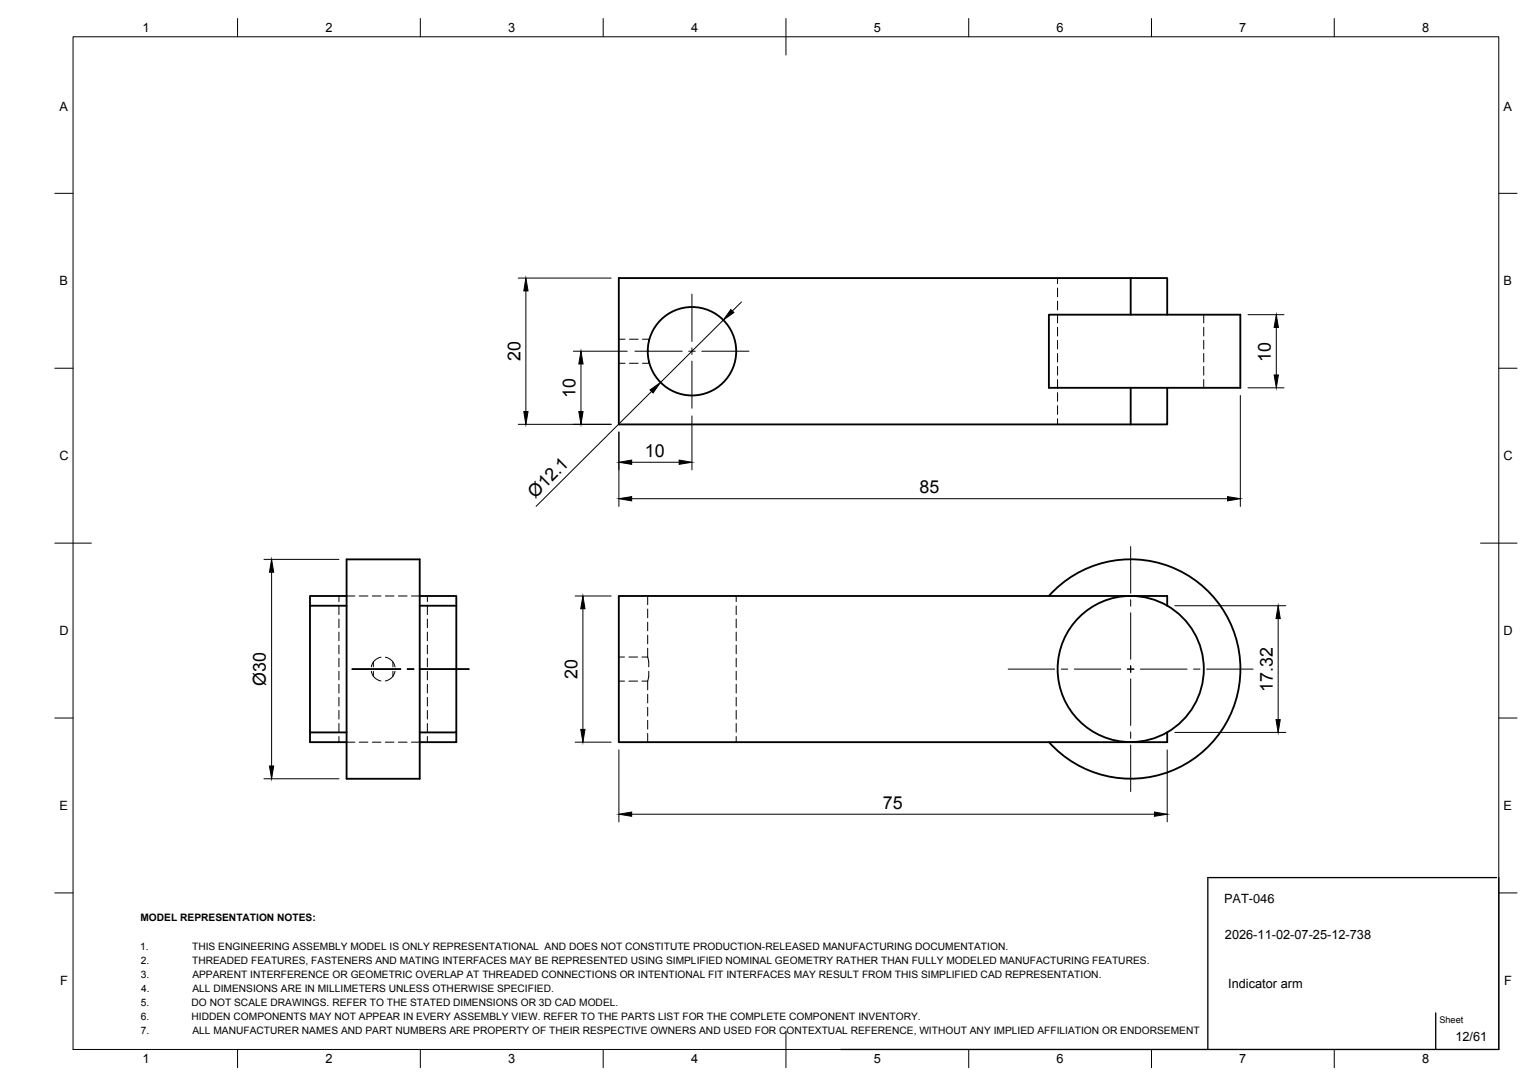
ISO-10303-21;
HEADER;
/* Generated by software containing ST-Developer
 * from STEP Tools, Inc. (www.steptools.com) 
 */

FILE_DESCRIPTION(
/* description */ ('Gear mesh backlash fixture'),
/* implementation_level */ '2;1');

FILE_NAME(
/* name */ 'Indicator arm.step',
/* time_stamp */ '2026-10-28T03:26:00-07:00',
/* author */ (''),
/* organization */ (''),
/* preprocessor_version */ 'ST-DEVELOPER v20.2',
/* originating_system */ 'Autodesk Translation Framework v15.17.0.0',
/* authorisation */ '');

FILE_SCHEMA (('AUTOMOTIVE_DESIGN { 1 0 10303 214 3 1 1 }'));
ENDSEC;

DATA;
#10=MECHANICAL_DESIGN_GEOMETRIC_PRESENTATION_REPRESENTATION('',(#1023),#57900);
#788=B_SPLINE_CURVE_WITH_KNOTS('',3,(#19722,#19723,#19724,#19725,#19726,
#19727,#19728,#19729,#19730,#19731,#19732,#19733,#19734,#19735),
 .UNSPECIFIED.,.F.,.F.,(4,2,2,2,2,2,4),(0.598759573717661,0.624973342427789,
0.687463163426142,0.749952984424494,0.812442805422847,0.874932626421199,
0.901146395131325),.UNSPECIFIED.);
#789=B_SPLINE_CURVE_WITH_KNOTS('',3,(#19739,#19740,#19741,#19742,#19743,
#19744,#19745,#19746),.UNSPECIFIED.,.F.,.F.,(4,2,2,4),(0.249984328141498,
0.31247414913985,0.374963970138203,0.401177738848332),.UNSPECIFIED.);
#790=B_SPLINE_CURVE_WITH_KNOTS('',3,(#19750,#19751,#19752,#19753,#19754,
#19755,#19756,#19757),.UNSPECIFIED.,.F.,.F.,(4,2,2,4),(0.0987909174346634,
0.125004686144793,0.187494507143146,0.249984328141498),.UNSPECIFIED.);
#923=SHAPE_REPRESENTATION_RELATIONSHIP('SRR','None',#58118,#973);
#973=ADVANCED_BREP_SHAPE_REPRESENTATION('',(#1088),#57851);
#1023=STYLED_ITEM('',(#58451),#1088);
#1088=MANIFOLD_SOLID_BREP('Body1',#13583);
#1199=FACE_BOUND('',#2617,.T.);
#1200=FACE_BOUND('',#2619,.T.);
#1201=FACE_BOUND('',#2625,.T.);
#1202=FACE_BOUND('',#2628,.T.);
#1368=PLANE('',#14390);
#1369=PLANE('',#14395);
#1370=PLANE('',#14407);
#1371=PLANE('',#14409);
#1372=PLANE('',#14410);
#1373=PLANE('',#14411);
#1374=PLANE('',#14412);
#1375=PLANE('',#14413);
#1376=PLANE('',#14414);
#1377=PLANE('',#14415);
#1378=PLANE('',#14416);
#1379=PLANE('',#14417);
#1380=PLANE('',#14418);
#1381=PLANE('',#14419);
#1382=PLANE('',#14420);
#1383=PLANE('',#14426);
#1384=PLANE('',#14427);
#1385=PLANE('',#14428);
#1386=PLANE('',#14429);
#1387=PLANE('',#14430);
#1388=PLANE('',#14431);
#1779=FACE_OUTER_BOUND('',#2600,.T.);
#1780=FACE_OUTER_BOUND('',#2601,.T.);
#1781=FACE_OUTER_BOUND('',#2602,.T.);
#1782=FACE_OUTER_BOUND('',#2603,.T.);
#1783=FACE_OUTER_BOUND('',#2604,.T.);
#1784=FACE_OUTER_BOUND('',#2605,.T.);
#1785=FACE_OUTER_BOUND('',#2606,.T.);
#1786=FACE_OUTER_BOUND('',#2607,.T.);
#1787=FACE_OUTER_BOUND('',#2608,.T.);
#1788=FACE_OUTER_BOUND('',#2609,.T.);
#1789=FACE_OUTER_BOUND('',#2610,.T.);
#1790=FACE_OUTER_BOUND('',#2611,.T.);
#1791=FACE_OUTER_BOUND('',#2612,.T.);
#1792=FACE_OUTER_BOUND('',#2613,.T.);
#1793=FACE_OUTER_BOUND('',#2614,.T.);
#1794=FACE_OUTER_BOUND('',#2615,.T.);
#1795=FACE_OUTER_BOUND('',#2616,.T.);
#1796=FACE_OUTER_BOUND('',#2618,.T.);
#1797=FACE_OUTER_BOUND('',#2620,.T.);
#1798=FACE_OUTER_BOUND('',#2621,.T.);
#1799=FACE_OUTER_BOUND('',#2622,.T.);
#1800=FACE_OUTER_BOUND('',#2623,.T.);
#1801=FACE_OUTER_BOUND('',#2624,.T.);
#1802=FACE_OUTER_BOUND('',#2626,.T.);
#1803=FACE_OUTER_BOUND('',#2627,.T.);
#2600=EDGE_LOOP('',(#9261,#9262));
#2601=EDGE_LOOP('',(#9263,#9264,#9265,#9266,#9267,#9268,#9269,#9270));
#2602=EDGE_LOOP('',(#9271,#9272));
#2603=EDGE_LOOP('',(#9273,#9274,#9275,#9276,#9277,#9278,#9279,#9280,#9281,
#9282,#9283,#9284,#9285,#9286,#9287,#9288,#9289,#9290,#9291,#9292,#9293,
#9294,#9295,#9296));
#2604=EDGE_LOOP('',(#9297,#9298,#9299,#9300,#9301,#9302,#9303,#9304,#9305));
#2605=EDGE_LOOP('',(#9306,#9307,#9308,#9309));
#2606=EDGE_LOOP('',(#9310,#9311,#9312));
#2607=EDGE_LOOP('',(#9313,#9314,#9315,#9316));
#2608=EDGE_LOOP('',(#9317,#9318,#9319,#9320));
#2609=EDGE_LOOP('',(#9321,#9322,#9323,#9324));
#2610=EDGE_LOOP('',(#9325,#9326,#9327,#9328));
#2611=EDGE_LOOP('',(#9329,#9330,#9331,#9332));
#2612=EDGE_LOOP('',(#9333,#9334,#9335,#9336));
#2613=EDGE_LOOP('',(#9337,#9338,#9339));
#2614=EDGE_LOOP('',(#9340,#9341,#9342));
#2615=EDGE_LOOP('',(#9343,#9344,#9345,#9346));
#2616=EDGE_LOOP('',(#9347,#9348,#9349,#9350,#9351,#9352,#9353,#9354));
#2617=EDGE_LOOP('',(#9355));
#2618=EDGE_LOOP('',(#9356,#9357,#9358,#9359));
#2619=EDGE_LOOP('',(#9360,#9361,#9362,#9363,#9364));
#2620=EDGE_LOOP('',(#9365,#9366,#9367,#9368));
#2621=EDGE_LOOP('',(#9369,#9370,#9371,#9372,#9373,#9374,#9375,#9376,#9377));
#2622=EDGE_LOOP('',(#9378,#9379,#9380,#9381));
#2623=EDGE_LOOP('',(#9382,#9383,#9384,#9385));
#2624=EDGE_LOOP('',(#9386,#9387,#9388,#9389));
#2625=EDGE_LOOP('',(#9390));
#2626=EDGE_LOOP('',(#9391,#9392,#9393));
#2627=EDGE_LOOP('',(#9394,#9395,#9396,#9397,#9398,#9399,#9400,#9401));
#2628=EDGE_LOOP('',(#9402));
#3498=LINE('',#19718,#4387);
#3499=LINE('',#19748,#4388);
#3500=LINE('',#19759,#4389);
#3501=LINE('',#19763,#4390);
#3502=LINE('',#19767,#4391);
#3503=LINE('',#19771,#4392);
#3504=LINE('',#19775,#4393);
#3505=LINE('',#19779,#4394);
#3506=LINE('',#19780,#4395);
#3507=LINE('',#19784,#4396);
#3508=LINE('',#19785,#4397);
#3509=LINE('',#19789,#4398);
#3510=LINE('',#19794,#4399);
#3511=LINE('',#19798,#4400);
#3512=LINE('',#19799,#4401);
#3513=LINE('',#19801,#4402);
#3514=LINE('',#19804,#4403);
#3515=LINE('',#19805,#4404);
#3516=LINE('',#19807,#4405);
#3517=LINE('',#19810,#4406);
#3518=LINE('',#19812,#4407);
#3519=LINE('',#19813,#4408);
#3520=LINE('',#19816,#4409);
#3521=LINE('',#19817,#4410);
#3522=LINE('',#19819,#4411);
#3523=LINE('',#19822,#4412);
#3524=LINE('',#19824,#4413);
#3525=LINE('',#19825,#4414);
#3526=LINE('',#19828,#4415);
#3527=LINE('',#19830,#4416);
#3528=LINE('',#19831,#4417);
#3529=LINE('',#19834,#4418);
#3530=LINE('',#19835,#4419);
#3531=LINE('',#19838,#4420);
#3532=LINE('',#19840,#4421);
#3533=LINE('',#19841,#4422);
#3534=LINE('',#19843,#4423);
#3535=LINE('',#19844,#4424);
#3536=LINE('',#19847,#4425);
#3537=LINE('',#19849,#4426);
#3538=LINE('',#19850,#4427);
#3539=LINE('',#19852,#4428);
#3540=LINE('',#19855,#4429);
#3541=LINE('',#19857,#4430);
#3542=LINE('',#19859,#4431);
#3543=LINE('',#19860,#4432);
#3544=LINE('',#19866,#4433);
#3545=LINE('',#19869,#4434);
#3546=LINE('',#19872,#4435);
#3547=LINE('',#19875,#4436);
#3548=LINE('',#19877,#4437);
#4387=VECTOR('',#16057,1.);
#4388=VECTOR('',#16064,0.164999999999999);
#4389=VECTOR('',#16069,1.);
#4390=VECTOR('',#16072,1.);
#4391=VECTOR('',#16075,1.);
#4392=VECTOR('',#16078,1.);
#4393=VECTOR('',#16081,1.);
#4394=VECTOR('',#16084,1.);
#4395=VECTOR('',#16085,1.);
#4396=VECTOR('',#16088,1.);
#4397=VECTOR('',#16089,1.);
#4398=VECTOR('',#16092,1.);
#4399=VECTOR('',#16097,1.);
#4400=VECTOR('',#16100,1.);
#4401=VECTOR('',#16101,1.);
#4402=VECTOR('',#16104,1.);
#4403=VECTOR('',#16107,1.);
#4404=VECTOR('',#16108,1.);
#4405=VECTOR('',#16109,1.);
#4406=VECTOR('',#16112,1.);
#4407=VECTOR('',#16113,1.);
#4408=VECTOR('',#16114,1.);
#4409=VECTOR('',#16117,1.);
#4410=VECTOR('',#16118,1.);
#4411=VECTOR('',#16121,1.);
#4412=VECTOR('',#16124,1.);
#4413=VECTOR('',#16125,1.);
#4414=VECTOR('',#16126,1.);
#4415=VECTOR('',#16129,1.);
#4416=VECTOR('',#16130,1.);
#4417=VECTOR('',#16131,1.);
#4418=VECTOR('',#16134,1.);
#4419=VECTOR('',#16135,1.);
#4420=VECTOR('',#16138,1.);
#4421=VECTOR('',#16139,1.);
#4422=VECTOR('',#16140,1.);
#4423=VECTOR('',#16143,1.);
#4424=VECTOR('',#16144,1.);
#4425=VECTOR('',#16147,1.);
#4426=VECTOR('',#16148,1.);
#4427=VECTOR('',#16149,1.);
#4428=VECTOR('',#16152,1.);
#4429=VECTOR('',#16157,1.);
#4430=VECTOR('',#16160,1.);
#4431=VECTOR('',#16161,1.);
#4432=VECTOR('',#16162,1.);
#4433=VECTOR('',#16169,0.605);
#4434=VECTOR('',#16172,1.);
#4435=VECTOR('',#16177,1.);
#4436=VECTOR('',#16182,1.);
#4437=VECTOR('',#16185,1.);
#5289=CIRCLE('',#14391,0.164999999999999);
#5290=CIRCLE('',#14393,0.164999999999999);
#5291=CIRCLE('',#14394,0.164999999999999);
#5292=CIRCLE('',#14397,1.);
#5293=CIRCLE('',#14398,1.);
#5294=CIRCLE('',#14399,1.);
#5295=CIRCLE('',#14400,1.);
#5296=CIRCLE('',#14401,1.);
#5297=CIRCLE('',#14402,1.);
#5298=CIRCLE('',#14403,1.);
#5299=CIRCLE('',#14404,1.);
#5300=CIRCLE('',#14405,1.);
#5301=CIRCLE('',#14406,1.);
#5302=CIRCLE('',#14408,1.5);
#5303=CIRCLE('',#14421,0.605);
#5304=CIRCLE('',#14423,0.605);
#5305=CIRCLE('',#14425,1.5);
#5909=VERTEX_POINT('',#19716);
#5910=VERTEX_POINT('',#19717);
#5911=VERTEX_POINT('',#19721);
#5912=VERTEX_POINT('',#19736);
#5913=VERTEX_POINT('',#19738);
#5914=VERTEX_POINT('',#19747);
#5915=VERTEX_POINT('',#19761);
#5916=VERTEX_POINT('',#19762);
#5917=VERTEX_POINT('',#19764);
#5918=VERTEX_POINT('',#19766);
#5919=VERTEX_POINT('',#19768);
#5920=VERTEX_POINT('',#19770);
#5921=VERTEX_POINT('',#19772);
#5922=VERTEX_POINT('',#19774);
#5923=VERTEX_POINT('',#19776);
#5924=VERTEX_POINT('',#19778);
#5925=VERTEX_POINT('',#19781);
#5926=VERTEX_POINT('',#19783);
#5927=VERTEX_POINT('',#19786);
#5928=VERTEX_POINT('',#19788);
#5929=VERTEX_POINT('',#19791);
#5930=VERTEX_POINT('',#19793);
#5931=VERTEX_POINT('',#19795);
#5932=VERTEX_POINT('',#19797);
#5933=VERTEX_POINT('',#19803);
#5934=VERTEX_POINT('',#19806);
#5935=VERTEX_POINT('',#19808);
#5936=VERTEX_POINT('',#19811);
#5937=VERTEX_POINT('',#19815);
#5938=VERTEX_POINT('',#19821);
#5939=VERTEX_POINT('',#19823);
#5940=VERTEX_POINT('',#19827);
#5941=VERTEX_POINT('',#19829);
#5942=VERTEX_POINT('',#19833);
#5943=VERTEX_POINT('',#19837);
#5944=VERTEX_POINT('',#19839);
#5945=VERTEX_POINT('',#19846);
#5946=VERTEX_POINT('',#19848);
#5947=VERTEX_POINT('',#19858);
#5948=VERTEX_POINT('',#19861);
#5949=VERTEX_POINT('',#19864);
#5950=VERTEX_POINT('',#19868);
#7217=EDGE_CURVE('',#5909,#5910,#3498,.T.);
#7218=EDGE_CURVE('',#5909,#5910,#5289,.T.);
#7219=EDGE_CURVE('',#5911,#5909,#788,.T.);
#7220=EDGE_CURVE('',#5912,#5911,#5290,.T.);
#7221=EDGE_CURVE('',#5913,#5912,#789,.T.);
#7222=EDGE_CURVE('',#5913,#5914,#3499,.T.);
#7223=EDGE_CURVE('',#5914,#5914,#5291,.T.);
#7224=EDGE_CURVE('',#5910,#5913,#790,.T.);
#7225=EDGE_CURVE('',#5912,#5911,#3500,.T.);
#7226=EDGE_CURVE('',#5915,#5916,#3501,.T.);
#7227=EDGE_CURVE('',#5917,#5915,#5292,.T.);
#7228=EDGE_CURVE('',#5918,#5917,#3502,.T.);
#7229=EDGE_CURVE('',#5919,#5918,#5293,.T.);
#7230=EDGE_CURVE('',#5919,#5920,#3503,.T.);
#7231=EDGE_CURVE('',#5921,#5920,#5294,.T.);
#7232=EDGE_CURVE('',#5922,#5921,#3504,.T.);
#7233=EDGE_CURVE('',#5923,#5922,#5295,.T.);
#7234=EDGE_CURVE('',#5924,#5923,#3505,.T.);
#7235=EDGE_CURVE('',#5924,#5923,#3506,.T.);
#7236=EDGE_CURVE('',#5925,#5923,#5296,.T.);
#7237=EDGE_CURVE('',#5926,#5925,#3507,.T.);
#7238=EDGE_CURVE('',#5926,#5925,#3508,.T.);
#7239=EDGE_CURVE('',#5927,#5925,#5297,.T.);
#7240=EDGE_CURVE('',#5928,#5927,#3509,.T.);
#7241=EDGE_CURVE('',#5920,#5928,#5298,.T.);
#7242=EDGE_CURVE('',#5929,#5919,#5299,.T.);
#7243=EDGE_CURVE('',#5930,#5929,#3510,.T.);
#7244=EDGE_CURVE('',#5931,#5930,#5300,.T.);
#7245=EDGE_CURVE('',#5931,#5932,#3511,.T.);
#7246=EDGE_CURVE('',#5931,#5932,#3512,.T.);
#7247=EDGE_CURVE('',#5915,#5931,#5301,.T.);
#7248=EDGE_CURVE('',#5915,#5916,#3513,.T.);
#7249=EDGE_CURVE('',#5933,#5918,#3514,.T.);
#7250=EDGE_CURVE('',#5916,#5933,#3515,.T.);
#7251=EDGE_CURVE('',#5934,#5916,#3516,.T.);
#7252=EDGE_CURVE('',#5935,#5934,#5302,.T.);
#7253=EDGE_CURVE('',#5932,#5935,#3517,.T.);
#7254=EDGE_CURVE('',#5936,#5932,#3518,.T.);
#7255=EDGE_CURVE('',#5929,#5936,#3519,.T.);
#7256=EDGE_CURVE('',#5917,#5937,#3520,.T.);
#7257=EDGE_CURVE('',#5933,#5937,#3521,.T.);
#7258=EDGE_CURVE('',#5937,#5915,#3522,.T.);
#7259=EDGE_CURVE('',#5931,#5938,#3523,.T.);
#7260=EDGE_CURVE('',#5938,#5939,#3524,.T.);
#7261=EDGE_CURVE('',#5915,#5939,#3525,.T.);
#7262=EDGE_CURVE('',#5926,#5940,#3526,.T.);
#7263=EDGE_CURVE('',#5941,#5940,#3527,.T.);
#7264=EDGE_CURVE('',#5925,#5941,#3528,.T.);
#7265=EDGE_CURVE('',#5942,#5931,#3529,.T.);
#7266=EDGE_CURVE('',#5936,#5942,#3530,.T.);
#7267=EDGE_CURVE('',#5921,#5943,#3531,.T.);
#7268=EDGE_CURVE('',#5944,#5943,#3532,.T.);
#7269=EDGE_CURVE('',#5922,#5944,#3533,.T.);
#7270=EDGE_CURVE('',#5941,#5927,#3534,.T.);
#7271=EDGE_CURVE('',#5940,#5928,#3535,.T.);
#7272=EDGE_CURVE('',#5945,#5923,#3536,.T.);
#7273=EDGE_CURVE('',#5946,#5945,#3537,.T.);
#7274=EDGE_CURVE('',#5946,#5925,#3538,.T.);
#7275=EDGE_CURVE('',#5923,#5944,#3539,.T.);
#7276=EDGE_CURVE('',#5943,#5924,#3540,.T.);
#7277=EDGE_CURVE('',#5939,#5945,#3541,.T.);
#7278=EDGE_CURVE('',#5924,#5947,#3542,.T.);
#7279=EDGE_CURVE('',#5947,#5934,#3543,.T.);
#7280=EDGE_CURVE('',#5948,#5948,#5303,.T.);
#7281=EDGE_CURVE('',#5949,#5949,#5304,.T.);
#7282=EDGE_CURVE('',#5949,#5948,#3544,.T.);
#7283=EDGE_CURVE('',#5935,#5950,#3545,.T.);
#7284=EDGE_CURVE('',#5950,#5947,#5305,.T.);
#7285=EDGE_CURVE('',#5950,#5926,#3546,.T.);
#7286=EDGE_CURVE('',#5942,#5930,#3547,.T.);
#7287=EDGE_CURVE('',#5938,#5946,#3548,.T.);
#9261=ORIENTED_EDGE('',*,*,#7217,.F.);
#9262=ORIENTED_EDGE('',*,*,#7218,.T.);
#9263=ORIENTED_EDGE('',*,*,#7219,.F.);
#9264=ORIENTED_EDGE('',*,*,#7220,.F.);
#9265=ORIENTED_EDGE('',*,*,#7221,.F.);
#9266=ORIENTED_EDGE('',*,*,#7222,.T.);
#9267=ORIENTED_EDGE('',*,*,#7223,.F.);
#9268=ORIENTED_EDGE('',*,*,#7222,.F.);
#9269=ORIENTED_EDGE('',*,*,#7224,.F.);
#9270=ORIENTED_EDGE('',*,*,#7218,.F.);
#9271=ORIENTED_EDGE('',*,*,#7225,.F.);
#9272=ORIENTED_EDGE('',*,*,#7220,.T.);
#9273=ORIENTED_EDGE('',*,*,#7226,.F.);
#9274=ORIENTED_EDGE('',*,*,#7227,.F.);
#9275=ORIENTED_EDGE('',*,*,#7228,.F.);
#9276=ORIENTED_EDGE('',*,*,#7229,.F.);
#9277=ORIENTED_EDGE('',*,*,#7230,.T.);
#9278=ORIENTED_EDGE('',*,*,#7231,.F.);
#9279=ORIENTED_EDGE('',*,*,#7232,.F.);
#9280=ORIENTED_EDGE('',*,*,#7233,.F.);
#9281=ORIENTED_EDGE('',*,*,#7234,.F.);
#9282=ORIENTED_EDGE('',*,*,#7235,.T.);
#9283=ORIENTED_EDGE('',*,*,#7236,.F.);
#9284=ORIENTED_EDGE('',*,*,#7237,.F.);
#9285=ORIENTED_EDGE('',*,*,#7238,.T.);
#9286=ORIENTED_EDGE('',*,*,#7239,.F.);
#9287=ORIENTED_EDGE('',*,*,#7240,.F.);
#9288=ORIENTED_EDGE('',*,*,#7241,.F.);
#9289=ORIENTED_EDGE('',*,*,#7230,.F.);
#9290=ORIENTED_EDGE('',*,*,#7242,.F.);
#9291=ORIENTED_EDGE('',*,*,#7243,.F.);
#9292=ORIENTED_EDGE('',*,*,#7244,.F.);
#9293=ORIENTED_EDGE('',*,*,#7245,.T.);
#9294=ORIENTED_EDGE('',*,*,#7246,.F.);
#9295=ORIENTED_EDGE('',*,*,#7247,.F.);
#9296=ORIENTED_EDGE('',*,*,#7248,.T.);
#9297=ORIENTED_EDGE('',*,*,#7242,.T.);
#9298=ORIENTED_EDGE('',*,*,#7229,.T.);
#9299=ORIENTED_EDGE('',*,*,#7249,.F.);
#9300=ORIENTED_EDGE('',*,*,#7250,.F.);
#9301=ORIENTED_EDGE('',*,*,#7251,.F.);
#9302=ORIENTED_EDGE('',*,*,#7252,.F.);
#9303=ORIENTED_EDGE('',*,*,#7253,.F.);
#9304=ORIENTED_EDGE('',*,*,#7254,.F.);
#9305=ORIENTED_EDGE('',*,*,#7255,.F.);
#9306=ORIENTED_EDGE('',*,*,#7228,.T.);
#9307=ORIENTED_EDGE('',*,*,#7256,.T.);
#9308=ORIENTED_EDGE('',*,*,#7257,.F.);
#9309=ORIENTED_EDGE('',*,*,#7249,.T.);
#9310=ORIENTED_EDGE('',*,*,#7227,.T.);
#9311=ORIENTED_EDGE('',*,*,#7258,.F.);
#9312=ORIENTED_EDGE('',*,*,#7256,.F.);
#9313=ORIENTED_EDGE('',*,*,#7247,.T.);
#9314=ORIENTED_EDGE('',*,*,#7259,.T.);
#9315=ORIENTED_EDGE('',*,*,#7260,.T.);
#9316=ORIENTED_EDGE('',*,*,#7261,.F.);
#9317=ORIENTED_EDGE('',*,*,#7238,.F.);
#9318=ORIENTED_EDGE('',*,*,#7262,.T.);
#9319=ORIENTED_EDGE('',*,*,#7263,.F.);
#9320=ORIENTED_EDGE('',*,*,#7264,.F.);
#9321=ORIENTED_EDGE('',*,*,#7245,.F.);
#9322=ORIENTED_EDGE('',*,*,#7265,.F.);
#9323=ORIENTED_EDGE('',*,*,#7266,.F.);
#9324=ORIENTED_EDGE('',*,*,#7254,.T.);
#9325=ORIENTED_EDGE('',*,*,#7232,.T.);
#9326=ORIENTED_EDGE('',*,*,#7267,.T.);
#9327=ORIENTED_EDGE('',*,*,#7268,.F.);
#9328=ORIENTED_EDGE('',*,*,#7269,.F.);
#9329=ORIENTED_EDGE('',*,*,#7240,.T.);
#9330=ORIENTED_EDGE('',*,*,#7270,.F.);
#9331=ORIENTED_EDGE('',*,*,#7263,.T.);
#9332=ORIENTED_EDGE('',*,*,#7271,.T.);
#9333=ORIENTED_EDGE('',*,*,#7236,.T.);
#9334=ORIENTED_EDGE('',*,*,#7272,.F.);
#9335=ORIENTED_EDGE('',*,*,#7273,.F.);
#9336=ORIENTED_EDGE('',*,*,#7274,.T.);
#9337=ORIENTED_EDGE('',*,*,#7233,.T.);
#9338=ORIENTED_EDGE('',*,*,#7269,.T.);
#9339=ORIENTED_EDGE('',*,*,#7275,.F.);
#9340=ORIENTED_EDGE('',*,*,#7239,.T.);
#9341=ORIENTED_EDGE('',*,*,#7264,.T.);
#9342=ORIENTED_EDGE('',*,*,#7270,.T.);
#9343=ORIENTED_EDGE('',*,*,#7234,.T.);
#9344=ORIENTED_EDGE('',*,*,#7275,.T.);
#9345=ORIENTED_EDGE('',*,*,#7268,.T.);
#9346=ORIENTED_EDGE('',*,*,#7276,.T.);
#9347=ORIENTED_EDGE('',*,*,#7248,.F.);
#9348=ORIENTED_EDGE('',*,*,#7261,.T.);
#9349=ORIENTED_EDGE('',*,*,#7277,.T.);
#9350=ORIENTED_EDGE('',*,*,#7272,.T.);
#9351=ORIENTED_EDGE('',*,*,#7235,.F.);
#9352=ORIENTED_EDGE('',*,*,#7278,.T.);
#9353=ORIENTED_EDGE('',*,*,#7279,.T.);
#9354=ORIENTED_EDGE('',*,*,#7251,.T.);
#9355=ORIENTED_EDGE('',*,*,#7280,.T.);
#9356=ORIENTED_EDGE('',*,*,#7281,.F.);
#9357=ORIENTED_EDGE('',*,*,#7282,.T.);
#9358=ORIENTED_EDGE('',*,*,#7280,.F.);
#9359=ORIENTED_EDGE('',*,*,#7282,.F.);
#9360=ORIENTED_EDGE('',*,*,#7224,.T.);
#9361=ORIENTED_EDGE('',*,*,#7221,.T.);
#9362=ORIENTED_EDGE('',*,*,#7225,.T.);
#9363=ORIENTED_EDGE('',*,*,#7219,.T.);
#9364=ORIENTED_EDGE('',*,*,#7217,.T.);
#9365=ORIENTED_EDGE('',*,*,#7283,.F.);
#9366=ORIENTED_EDGE('',*,*,#7252,.T.);
#9367=ORIENTED_EDGE('',*,*,#7279,.F.);
#9368=ORIENTED_EDGE('',*,*,#7284,.F.);
#9369=ORIENTED_EDGE('',*,*,#7231,.T.);
#9370=ORIENTED_EDGE('',*,*,#7241,.T.);
#9371=ORIENTED_EDGE('',*,*,#7271,.F.);
#9372=ORIENTED_EDGE('',*,*,#7262,.F.);
#9373=ORIENTED_EDGE('',*,*,#7285,.F.);
#9374=ORIENTED_EDGE('',*,*,#7284,.T.);
#9375=ORIENTED_EDGE('',*,*,#7278,.F.);
#9376=ORIENTED_EDGE('',*,*,#7276,.F.);
#9377=ORIENTED_EDGE('',*,*,#7267,.F.);
#9378=ORIENTED_EDGE('',*,*,#7226,.T.);
#9379=ORIENTED_EDGE('',*,*,#7250,.T.);
#9380=ORIENTED_EDGE('',*,*,#7257,.T.);
#9381=ORIENTED_EDGE('',*,*,#7258,.T.);
#9382=ORIENTED_EDGE('',*,*,#7243,.T.);
#9383=ORIENTED_EDGE('',*,*,#7255,.T.);
#9384=ORIENTED_EDGE('',*,*,#7266,.T.);
#9385=ORIENTED_EDGE('',*,*,#7286,.T.);
#9386=ORIENTED_EDGE('',*,*,#7287,.T.);
#9387=ORIENTED_EDGE('',*,*,#7273,.T.);
#9388=ORIENTED_EDGE('',*,*,#7277,.F.);
#9389=ORIENTED_EDGE('',*,*,#7260,.F.);
#9390=ORIENTED_EDGE('',*,*,#7223,.T.);
#9391=ORIENTED_EDGE('',*,*,#7244,.T.);
#9392=ORIENTED_EDGE('',*,*,#7286,.F.);
#9393=ORIENTED_EDGE('',*,*,#7265,.T.);
#9394=ORIENTED_EDGE('',*,*,#7246,.T.);
#9395=ORIENTED_EDGE('',*,*,#7253,.T.);
#9396=ORIENTED_EDGE('',*,*,#7283,.T.);
#9397=ORIENTED_EDGE('',*,*,#7285,.T.);
#9398=ORIENTED_EDGE('',*,*,#7237,.T.);
#9399=ORIENTED_EDGE('',*,*,#7274,.F.);
#9400=ORIENTED_EDGE('',*,*,#7287,.F.);
#9401=ORIENTED_EDGE('',*,*,#7259,.F.);
#9402=ORIENTED_EDGE('',*,*,#7281,.T.);
#12632=CYLINDRICAL_SURFACE('',#14392,0.164999999999999);
#12633=CYLINDRICAL_SURFACE('',#14396,1.);
#12634=CYLINDRICAL_SURFACE('',#14422,0.605);
#12635=CYLINDRICAL_SURFACE('',#14424,1.5);
#12896=ADVANCED_FACE('',(#1779),#1368,.T.);
#12897=ADVANCED_FACE('',(#1780),#12632,.F.);
#12898=ADVANCED_FACE('',(#1781),#1369,.T.);
#12899=ADVANCED_FACE('',(#1782),#12633,.F.);
#12900=ADVANCED_FACE('',(#1783),#1370,.F.);
#12901=ADVANCED_FACE('',(#1784),#1371,.T.);
#12902=ADVANCED_FACE('',(#1785),#1372,.T.);
#12903=ADVANCED_FACE('',(#1786),#1373,.T.);
#12904=ADVANCED_FACE('',(#1787),#1374,.F.);
#12905=ADVANCED_FACE('',(#1788),#1375,.F.);
#12906=ADVANCED_FACE('',(#1789),#1376,.T.);
#12907=ADVANCED_FACE('',(#1790),#1377,.T.);
#12908=ADVANCED_FACE('',(#1791),#1378,.T.);
#12909=ADVANCED_FACE('',(#1792),#1379,.T.);
#12910=ADVANCED_FACE('',(#1793),#1380,.T.);
#12911=ADVANCED_FACE('',(#1794),#1381,.T.);
#12912=ADVANCED_FACE('',(#1795,#1199),#1382,.T.);
#12913=ADVANCED_FACE('',(#1796,#1200),#12634,.F.);
#12914=ADVANCED_FACE('',(#1797),#12635,.T.);
#12915=ADVANCED_FACE('',(#1798),#1383,.T.);
#12916=ADVANCED_FACE('',(#1799),#1384,.T.);
#12917=ADVANCED_FACE('',(#1800),#1385,.T.);
#12918=ADVANCED_FACE('',(#1801,#1201),#1386,.T.);
#12919=ADVANCED_FACE('',(#1802),#1387,.T.);
#12920=ADVANCED_FACE('',(#1803,#1202),#1388,.F.);
#13583=CLOSED_SHELL('',(#12896,#12897,#12898,#12899,#12900,#12901,#12902,
#12903,#12904,#12905,#12906,#12907,#12908,#12909,#12910,#12911,#12912,#12913,
#12914,#12915,#12916,#12917,#12918,#12919,#12920));
#14389=AXIS2_PLACEMENT_3D('',#19714,#16053,#16054);
#14390=AXIS2_PLACEMENT_3D('',#19715,#16055,#16056);
#14391=AXIS2_PLACEMENT_3D('',#19719,#16058,#16059);
#14392=AXIS2_PLACEMENT_3D('',#19720,#16060,#16061);
#14393=AXIS2_PLACEMENT_3D('',#19737,#16062,#16063);
#14394=AXIS2_PLACEMENT_3D('',#19749,#16065,#16066);
#14395=AXIS2_PLACEMENT_3D('',#19758,#16067,#16068);
#14396=AXIS2_PLACEMENT_3D('',#19760,#16070,#16071);
#14397=AXIS2_PLACEMENT_3D('',#19765,#16073,#16074);
#14398=AXIS2_PLACEMENT_3D('',#19769,#16076,#16077);
#14399=AXIS2_PLACEMENT_3D('',#19773,#16079,#16080);
#14400=AXIS2_PLACEMENT_3D('',#19777,#16082,#16083);
#14401=AXIS2_PLACEMENT_3D('',#19782,#16086,#16087);
#14402=AXIS2_PLACEMENT_3D('',#19787,#16090,#16091);
#14403=AXIS2_PLACEMENT_3D('',#19790,#16093,#16094);
#14404=AXIS2_PLACEMENT_3D('',#19792,#16095,#16096);
#14405=AXIS2_PLACEMENT_3D('',#19796,#16098,#16099);
#14406=AXIS2_PLACEMENT_3D('',#19800,#16102,#16103);
#14407=AXIS2_PLACEMENT_3D('',#19802,#16105,#16106);
#14408=AXIS2_PLACEMENT_3D('',#19809,#16110,#16111);
#14409=AXIS2_PLACEMENT_3D('',#19814,#16115,#16116);
#14410=AXIS2_PLACEMENT_3D('',#19818,#16119,#16120);
#14411=AXIS2_PLACEMENT_3D('',#19820,#16122,#16123);
#14412=AXIS2_PLACEMENT_3D('',#19826,#16127,#16128);
#14413=AXIS2_PLACEMENT_3D('',#19832,#16132,#16133);
#14414=AXIS2_PLACEMENT_3D('',#19836,#16136,#16137);
#14415=AXIS2_PLACEMENT_3D('',#19842,#16141,#16142);
#14416=AXIS2_PLACEMENT_3D('',#19845,#16145,#16146);
#14417=AXIS2_PLACEMENT_3D('',#19851,#16150,#16151);
#14418=AXIS2_PLACEMENT_3D('',#19853,#16153,#16154);
#14419=AXIS2_PLACEMENT_3D('',#19854,#16155,#16156);
#14420=AXIS2_PLACEMENT_3D('',#19856,#16158,#16159);
#14421=AXIS2_PLACEMENT_3D('',#19862,#16163,#16164);
#14422=AXIS2_PLACEMENT_3D('',#19863,#16165,#16166);
#14423=AXIS2_PLACEMENT_3D('',#19865,#16167,#16168);
#14424=AXIS2_PLACEMENT_3D('',#19867,#16170,#16171);
#14425=AXIS2_PLACEMENT_3D('',#19870,#16173,#16174);
#14426=AXIS2_PLACEMENT_3D('',#19871,#16175,#16176);
#14427=AXIS2_PLACEMENT_3D('',#19873,#16178,#16179);
#14428=AXIS2_PLACEMENT_3D('',#19874,#16180,#16181);
#14429=AXIS2_PLACEMENT_3D('',#19876,#16183,#16184);
#14430=AXIS2_PLACEMENT_3D('',#19878,#16186,#16187);
#14431=AXIS2_PLACEMENT_3D('',#19879,#16188,#16189);
#16053=DIRECTION('axis',(0.,0.,1.));
#16054=DIRECTION('refdir',(1.,0.,0.));
#16055=DIRECTION('center_axis',(1.,0.,0.));
#16056=DIRECTION('ref_axis',(0.,0.,-1.));
#16057=DIRECTION('',(0.,0.,1.));
#16058=DIRECTION('center_axis',(1.,0.,0.));
#16059=DIRECTION('ref_axis',(0.,0.,-1.));
#16060=DIRECTION('center_axis',(1.,0.,0.));
#16061=DIRECTION('ref_axis',(0.,0.,-1.));
#16062=DIRECTION('center_axis',(1.,0.,0.));
#16063=DIRECTION('ref_axis',(0.,0.,-1.));
#16064=DIRECTION('',(1.,0.,0.));
#16065=DIRECTION('center_axis',(-1.,0.,0.));
#16066=DIRECTION('ref_axis',(0.,0.,-1.));
#16067=DIRECTION('center_axis',(1.,0.,0.));
#16068=DIRECTION('ref_axis',(0.,0.,-1.));
#16069=DIRECTION('',(0.,0.,-1.));
#16070=DIRECTION('center_axis',(0.,1.,0.));
#16071=DIRECTION('ref_axis',(1.,0.,0.));
#16072=DIRECTION('',(0.,1.,0.));
#16073=DIRECTION('center_axis',(0.,1.,0.));
#16074=DIRECTION('ref_axis',(1.,0.,0.));
#16075=DIRECTION('',(0.,-1.,0.));
#16076=DIRECTION('center_axis',(0.,1.,0.));
#16077=DIRECTION('ref_axis',(1.,0.,0.));
#16078=DIRECTION('',(0.,1.,0.));
#16079=DIRECTION('center_axis',(0.,-1.,0.));
#16080=DIRECTION('ref_axis',(1.,0.,0.));
#16081=DIRECTION('',(0.,-1.,0.));
#16082=DIRECTION('center_axis',(0.,-1.,0.));
#16083=DIRECTION('ref_axis',(1.,0.,0.));
#16084=DIRECTION('',(0.,1.,0.));
#16085=DIRECTION('',(0.,1.,0.));
#16086=DIRECTION('center_axis',(0.,-1.,0.));
#16087=DIRECTION('ref_axis',(1.,0.,0.));
#16088=DIRECTION('',(0.,1.,0.));
#16089=DIRECTION('',(0.,1.,0.));
#16090=DIRECTION('center_axis',(0.,-1.,0.));
#16091=DIRECTION('ref_axis',(1.,0.,0.));
#16092=DIRECTION('',(0.,1.,0.));
#16093=DIRECTION('center_axis',(0.,-1.,0.));
#16094=DIRECTION('ref_axis',(1.,0.,0.));
#16095=DIRECTION('center_axis',(0.,1.,0.));
#16096=DIRECTION('ref_axis',(1.,0.,0.));
#16097=DIRECTION('',(0.,1.,0.));
#16098=DIRECTION('center_axis',(0.,1.,0.));
#16099=DIRECTION('ref_axis',(1.,0.,0.));
#16100=DIRECTION('',(0.,1.,0.));
#16101=DIRECTION('',(0.,1.,0.));
#16102=DIRECTION('center_axis',(0.,1.,0.));
#16103=DIRECTION('ref_axis',(1.,0.,0.));
#16104=DIRECTION('',(0.,1.,0.));
#16105=DIRECTION('center_axis',(0.,1.,0.));
#16106=DIRECTION('ref_axis',(1.,0.,0.));
#16107=DIRECTION('',(0.,0.,-1.));
#16108=DIRECTION('',(-1.,0.,0.));
#16109=DIRECTION('',(-1.,0.,0.));
#16110=DIRECTION('center_axis',(0.,1.,0.));
#16111=DIRECTION('ref_axis',(1.,0.,0.));
#16112=DIRECTION('',(1.,0.,0.));
#16113=DIRECTION('',(1.,0.,0.));
#16114=DIRECTION('',(0.,0.,-1.));
#16115=DIRECTION('center_axis',(-1.,0.,0.));
#16116=DIRECTION('ref_axis',(0.,-1.,0.));
#16117=DIRECTION('',(0.,0.,1.));
#16118=DIRECTION('',(0.,-1.,0.));
#16119=DIRECTION('center_axis',(0.,-1.,0.));
#16120=DIRECTION('ref_axis',(1.,0.,0.));
#16121=DIRECTION('',(1.,0.,0.));
#16122=DIRECTION('center_axis',(0.,-1.,0.));
#16123=DIRECTION('ref_axis',(1.,0.,0.));
#16124=DIRECTION('',(1.,0.,0.));
#16125=DIRECTION('',(0.,0.,1.));
#16126=DIRECTION('',(1.,0.,0.));
#16127=DIRECTION('center_axis',(0.,0.,1.));
#16128=DIRECTION('ref_axis',(1.,0.,0.));
#16129=DIRECTION('',(-1.,0.,0.));
#16130=DIRECTION('',(0.,-1.,0.));
#16131=DIRECTION('',(-1.,0.,0.));
#16132=DIRECTION('center_axis',(0.,0.,1.));
#16133=DIRECTION('ref_axis',(1.,0.,0.));
#16134=DIRECTION('',(1.,0.,0.));
#16135=DIRECTION('',(0.,-1.,0.));
#16136=DIRECTION('center_axis',(-1.,0.,0.));
#16137=DIRECTION('ref_axis',(0.,-1.,0.));
#16138=DIRECTION('',(0.,0.,1.));
#16139=DIRECTION('',(0.,-1.,0.));
#16140=DIRECTION('',(0.,0.,1.));
#16141=DIRECTION('center_axis',(-1.,0.,0.));
#16142=DIRECTION('ref_axis',(0.,-1.,0.));
#16143=DIRECTION('',(0.,0.,1.));
#16144=DIRECTION('',(0.,0.,1.));
#16145=DIRECTION('center_axis',(0.,1.,0.));
#16146=DIRECTION('ref_axis',(-1.,0.,0.));
#16147=DIRECTION('',(-1.,0.,0.));
#16148=DIRECTION('',(0.,0.,1.));
#16149=DIRECTION('',(-1.,0.,0.));
#16150=DIRECTION('center_axis',(0.,1.,0.));
#16151=DIRECTION('ref_axis',(-1.,0.,0.));
#16152=DIRECTION('',(-1.,0.,0.));
#16153=DIRECTION('center_axis',(0.,1.,0.));
#16154=DIRECTION('ref_axis',(-1.,0.,0.));
#16155=DIRECTION('center_axis',(0.,0.,1.));
#16156=DIRECTION('ref_axis',(1.,0.,0.));
#16157=DIRECTION('',(1.,0.,0.));
#16158=DIRECTION('center_axis',(0.,0.,1.));
#16159=DIRECTION('ref_axis',(1.,0.,0.));
#16160=DIRECTION('',(0.,1.,0.));
#16161=DIRECTION('',(1.,0.,0.));
#16162=DIRECTION('',(0.,-1.,0.));
#16163=DIRECTION('center_axis',(0.,0.,-1.));
#16164=DIRECTION('ref_axis',(1.,0.,0.));
#16165=DIRECTION('center_axis',(0.,0.,1.));
#16166=DIRECTION('ref_axis',(1.,0.,0.));
#16167=DIRECTION('center_axis',(0.,0.,1.));
#16168=DIRECTION('ref_axis',(1.,0.,0.));
#16169=DIRECTION('',(0.,0.,1.));
#16170=DIRECTION('center_axis',(0.,1.,0.));
#16171=DIRECTION('ref_axis',(-1.,0.,-1.22464679914735E-16));
#16172=DIRECTION('',(0.,1.,0.));
#16173=DIRECTION('center_axis',(0.,1.,0.));
#16174=DIRECTION('ref_axis',(1.,0.,0.));
#16175=DIRECTION('center_axis',(0.,1.,0.));
#16176=DIRECTION('ref_axis',(1.,0.,0.));
#16177=DIRECTION('',(-1.,0.,0.));
#16178=DIRECTION('center_axis',(0.,0.,1.));
#16179=DIRECTION('ref_axis',(1.,0.,0.));
#16180=DIRECTION('center_axis',(-1.,0.,0.));
#16181=DIRECTION('ref_axis',(0.,-1.,0.));
#16182=DIRECTION('',(0.,0.,1.));
#16183=DIRECTION('center_axis',(1.,0.,0.));
#16184=DIRECTION('ref_axis',(0.,1.,0.));
#16185=DIRECTION('',(0.,1.,0.));
#16186=DIRECTION('center_axis',(0.,-1.,0.));
#16187=DIRECTION('ref_axis',(1.,0.,0.));
#16188=DIRECTION('center_axis',(0.,0.,1.));
#16189=DIRECTION('ref_axis',(1.,0.,0.));
#19714=CARTESIAN_POINT('',(0.,0.,0.));
#19715=CARTESIAN_POINT('Origin',(12.59,9.,12.));
#19716=CARTESIAN_POINT('',(12.59,9.13388427838995,11.9035634923901));
#19717=CARTESIAN_POINT('',(12.59,9.13388427838995,12.0964365076099));
#19718=CARTESIAN_POINT('',(12.59,9.13388427838995,10.9));
#19719=CARTESIAN_POINT('Origin',(12.59,9.,12.));
#19720=CARTESIAN_POINT('Origin',(12.59,9.,12.));
#19721=CARTESIAN_POINT('',(12.59,8.86611572161005,11.9035634923901));
#19722=CARTESIAN_POINT('Ctrl Pts',(12.59,8.86611572161005,11.9035634923901));
#19723=CARTESIAN_POINT('Ctrl Pts',(12.5911984034061,8.87139683465861,11.8962316423768));
#19724=CARTESIAN_POINT('Ctrl Pts',(12.5924406412882,8.87720755102006,11.8894472111884));
#19725=CARTESIAN_POINT('Ctrl Pts',(12.5965106411141,8.89791616804014,11.8687385941683));
#19726=CARTESIAN_POINT('Ctrl Pts',(12.5995440949832,8.91639978640534,11.8560565239921));
#19727=CARTESIAN_POINT('Ctrl Pts',(12.603817074383,8.95702258499573,11.8391843843662));
#19728=CARTESIAN_POINT('Ctrl Pts',(12.605,8.97917005966722,11.835));
#19729=CARTESIAN_POINT('Ctrl Pts',(12.605,9.02082994033278,11.835));
#19730=CARTESIAN_POINT('Ctrl Pts',(12.603817074383,9.04297741500427,11.8391843843662));
#19731=CARTESIAN_POINT('Ctrl Pts',(12.5995440949832,9.08360021359466,11.8560565239921));
#19732=CARTESIAN_POINT('Ctrl Pts',(12.5965106411141,9.10208383195986,11.8687385941683));
#19733=CARTESIAN_POINT('Ctrl Pts',(12.5924406412882,9.12279244897994,11.8894472111884));
#19734=CARTESIAN_POINT('Ctrl Pts',(12.5911984034061,9.12860316534139,11.8962316423768));
#19735=CARTESIAN_POINT('Ctrl Pts',(12.59,9.13388427838995,11.9035634923901));
#19736=CARTESIAN_POINT('',(12.59,8.86611572161005,12.0964365076099));
#19737=CARTESIAN_POINT('Origin',(12.59,9.,12.));
#19738=CARTESIAN_POINT('',(12.605,9.,12.165));
#19739=CARTESIAN_POINT('Ctrl Pts',(12.605,9.,12.165));
#19740=CARTESIAN_POINT('Ctrl Pts',(12.605,8.97917005966722,12.165));
#19741=CARTESIAN_POINT('Ctrl Pts',(12.603817074383,8.95702258499573,12.1608156156338));
#19742=CARTESIAN_POINT('Ctrl Pts',(12.5995440949832,8.91639978640534,12.1439434760079));
#19743=CARTESIAN_POINT('Ctrl Pts',(12.5965106411141,8.89791616804014,12.1312614058317));
#19744=CARTESIAN_POINT('Ctrl Pts',(12.5924406412882,8.87720755102006,12.1105527888116));
#19745=CARTESIAN_POINT('Ctrl Pts',(12.5911984034061,8.87139683465861,12.1037683576232));
#19746=CARTESIAN_POINT('Ctrl Pts',(12.59,8.86611572161005,12.0964365076099));
#19747=CARTESIAN_POINT('',(13.,9.,12.165));
#19748=CARTESIAN_POINT('',(12.59,9.,12.165));
#19749=CARTESIAN_POINT('Origin',(13.,9.,12.));
#19750=CARTESIAN_POINT('Ctrl Pts',(12.59,9.13388427838995,12.0964365076099));
#19751=CARTESIAN_POINT('Ctrl Pts',(12.5911984034061,9.12860316534139,12.1037683576232));
#19752=CARTESIAN_POINT('Ctrl Pts',(12.5924406412882,9.12279244897994,12.1105527888116));
#19753=CARTESIAN_POINT('Ctrl Pts',(12.5965106411141,9.10208383195986,12.1312614058317));
#19754=CARTESIAN_POINT('Ctrl Pts',(12.5995440949832,9.08360021359466,12.1439434760079));
#19755=CARTESIAN_POINT('Ctrl Pts',(12.603817074383,9.04297741500427,12.1608156156338));
#19756=CARTESIAN_POINT('Ctrl Pts',(12.605,9.02082994033278,12.165));
#19757=CARTESIAN_POINT('Ctrl Pts',(12.605,9.,12.165));
#19758=CARTESIAN_POINT('Origin',(12.59,9.,12.));
#19759=CARTESIAN_POINT('',(12.59,8.86611572161005,10.9));
#19760=CARTESIAN_POINT('Origin',(6.,7.9,12.));
#19761=CARTESIAN_POINT('',(6.,8.,13.));
#19762=CARTESIAN_POINT('',(6.,8.5,13.));
#19763=CARTESIAN_POINT('',(6.,7.9,13.));
#19764=CARTESIAN_POINT('',(5.5,8.,12.8660254037844));
#19765=CARTESIAN_POINT('Origin',(6.,8.,12.));
#19766=CARTESIAN_POINT('',(5.5,8.5,12.8660254037844));
#19767=CARTESIAN_POINT('',(5.5,7.9,12.8660254037844));
#19768=CARTESIAN_POINT('',(5.,8.5,12.));
#19769=CARTESIAN_POINT('Origin',(6.,8.5,12.));
#19770=CARTESIAN_POINT('',(5.,9.5,12.));
#19771=CARTESIAN_POINT('',(5.,7.9,12.));
#19772=CARTESIAN_POINT('',(5.5,9.5,12.8660254037844));
#19773=CARTESIAN_POINT('Origin',(6.,9.5,12.));
#19774=CARTESIAN_POINT('',(5.5,10.,12.8660254037844));
#19775=CARTESIAN_POINT('',(5.5,7.9,12.8660254037844));
#19776=CARTESIAN_POINT('',(6.,10.,13.));
#19777=CARTESIAN_POINT('Origin',(6.,10.,12.));
#19778=CARTESIAN_POINT('',(6.,9.5,13.));
#19779=CARTESIAN_POINT('',(6.,7.9,13.));
#19780=CARTESIAN_POINT('',(6.,7.9,13.));
#19781=CARTESIAN_POINT('',(6.,10.,11.));
#19782=CARTESIAN_POINT('Origin',(6.,10.,12.));
#19783=CARTESIAN_POINT('',(6.,9.5,11.));
#19784=CARTESIAN_POINT('',(6.,7.9,11.));
#19785=CARTESIAN_POINT('',(6.,7.9,11.));
#19786=CARTESIAN_POINT('',(5.5,10.,11.1339745962156));
#19787=CARTESIAN_POINT('Origin',(6.,10.,12.));
#19788=CARTESIAN_POINT('',(5.5,9.5,11.1339745962156));
#19789=CARTESIAN_POINT('',(5.5,7.9,11.1339745962156));
#19790=CARTESIAN_POINT('Origin',(6.,9.5,12.));
#19791=CARTESIAN_POINT('',(5.5,8.5,11.1339745962156));
#19792=CARTESIAN_POINT('Origin',(6.,8.5,12.));
#19793=CARTESIAN_POINT('',(5.5,8.,11.1339745962156));
#19794=CARTESIAN_POINT('',(5.5,7.9,11.1339745962156));
#19795=CARTESIAN_POINT('',(6.,8.,11.));
#19796=CARTESIAN_POINT('Origin',(6.,8.,12.));
#19797=CARTESIAN_POINT('',(6.,8.5,11.));
#19798=CARTESIAN_POINT('',(6.,7.9,11.));
#19799=CARTESIAN_POINT('',(6.,7.9,11.));
#19800=CARTESIAN_POINT('Origin',(6.,8.,12.));
#19801=CARTESIAN_POINT('',(6.,7.9,13.));
#19802=CARTESIAN_POINT('Origin',(6.,8.5,12.));
#19803=CARTESIAN_POINT('',(5.5,8.5,13.));
#19804=CARTESIAN_POINT('',(5.5,8.5,11.5));
#19805=CARTESIAN_POINT('',(7.625,8.5,13.));
#19806=CARTESIAN_POINT('',(7.11803398874989,8.5,13.));
#19807=CARTESIAN_POINT('',(7.625,8.5,13.));
#19808=CARTESIAN_POINT('',(7.11803398874989,8.5,11.));
#19809=CARTESIAN_POINT('Origin',(6.,8.5,12.));
#19810=CARTESIAN_POINT('',(7.625,8.5,11.));
#19811=CARTESIAN_POINT('',(5.5,8.5,11.));
#19812=CARTESIAN_POINT('',(7.625,8.5,11.));
#19813=CARTESIAN_POINT('',(5.5,8.5,11.5));
#19814=CARTESIAN_POINT('Origin',(5.5,10.,11.));
#19815=CARTESIAN_POINT('',(5.5,8.,13.));
#19816=CARTESIAN_POINT('',(5.5,8.,11.));
#19817=CARTESIAN_POINT('',(5.5,10.,13.));
#19818=CARTESIAN_POINT('Origin',(5.5,8.,11.));
#19819=CARTESIAN_POINT('',(5.5,8.,13.));
#19820=CARTESIAN_POINT('Origin',(5.5,8.,11.));
#19821=CARTESIAN_POINT('',(13.,8.,11.));
#19822=CARTESIAN_POINT('',(5.5,8.,11.));
#19823=CARTESIAN_POINT('',(13.,8.,13.));
#19824=CARTESIAN_POINT('',(13.,8.,11.));
#19825=CARTESIAN_POINT('',(5.5,8.,13.));
#19826=CARTESIAN_POINT('Origin',(9.25,9.,11.));
#19827=CARTESIAN_POINT('',(5.5,9.5,11.));
#19828=CARTESIAN_POINT('',(7.625,9.5,11.));
#19829=CARTESIAN_POINT('',(5.5,10.,11.));
#19830=CARTESIAN_POINT('',(5.5,10.,11.));
#19831=CARTESIAN_POINT('',(13.,10.,11.));
#19832=CARTESIAN_POINT('Origin',(9.25,9.,11.));
#19833=CARTESIAN_POINT('',(5.5,8.,11.));
#19834=CARTESIAN_POINT('',(5.5,8.,11.));
#19835=CARTESIAN_POINT('',(5.5,10.,11.));
#19836=CARTESIAN_POINT('Origin',(5.5,10.,11.));
#19837=CARTESIAN_POINT('',(5.5,9.5,13.));
#19838=CARTESIAN_POINT('',(5.5,9.5,11.5));
#19839=CARTESIAN_POINT('',(5.5,10.,13.));
#19840=CARTESIAN_POINT('',(5.5,10.,13.));
#19841=CARTESIAN_POINT('',(5.5,10.,11.));
#19842=CARTESIAN_POINT('Origin',(5.5,10.,11.));
#19843=CARTESIAN_POINT('',(5.5,10.,11.));
#19844=CARTESIAN_POINT('',(5.5,9.5,11.5));
#19845=CARTESIAN_POINT('Origin',(13.,10.,11.));
#19846=CARTESIAN_POINT('',(13.,10.,13.));
#19847=CARTESIAN_POINT('',(13.,10.,13.));
#19848=CARTESIAN_POINT('',(13.,10.,11.));
#19849=CARTESIAN_POINT('',(13.,10.,11.));
#19850=CARTESIAN_POINT('',(13.,10.,11.));
#19851=CARTESIAN_POINT('Origin',(13.,10.,11.));
#19852=CARTESIAN_POINT('',(13.,10.,13.));
#19853=CARTESIAN_POINT('Origin',(13.,10.,11.));
#19854=CARTESIAN_POINT('Origin',(9.25,9.,13.));
#19855=CARTESIAN_POINT('',(7.625,9.5,13.));
#19856=CARTESIAN_POINT('Origin',(9.25,9.,13.));
#19857=CARTESIAN_POINT('',(13.,8.,13.));
#19858=CARTESIAN_POINT('',(7.11803398874989,9.5,13.));
#19859=CARTESIAN_POINT('',(7.625,9.5,13.));
#19860=CARTESIAN_POINT('',(7.11803398874989,8.5,13.));
#19861=CARTESIAN_POINT('',(11.395,9.,13.));
#19862=CARTESIAN_POINT('Origin',(12.,9.,13.));
#19863=CARTESIAN_POINT('Origin',(12.,9.,10.9));
#19864=CARTESIAN_POINT('',(11.395,9.,11.));
#19865=CARTESIAN_POINT('Origin',(12.,9.,11.));
#19866=CARTESIAN_POINT('',(11.395,9.,10.9));
#19867=CARTESIAN_POINT('Origin',(6.,8.5,12.));
#19868=CARTESIAN_POINT('',(7.11803398874989,9.5,11.));
#19869=CARTESIAN_POINT('',(7.11803398874989,8.5,11.));
#19870=CARTESIAN_POINT('Origin',(6.,9.5,12.));
#19871=CARTESIAN_POINT('Origin',(6.,9.5,12.));
#19872=CARTESIAN_POINT('',(7.625,9.5,11.));
#19873=CARTESIAN_POINT('Origin',(9.25,9.,13.));
#19874=CARTESIAN_POINT('Origin',(5.5,10.,11.));
#19875=CARTESIAN_POINT('',(5.5,8.,11.));
#19876=CARTESIAN_POINT('Origin',(13.,8.,11.));
#19877=CARTESIAN_POINT('',(13.,8.,11.));
#19878=CARTESIAN_POINT('Origin',(5.5,8.,11.));
#19879=CARTESIAN_POINT('Origin',(9.25,9.,11.));
#57792=UNCERTAINTY_MEASURE_WITH_UNIT(LENGTH_MEASURE(0.001),#57901,
'DISTANCE_ACCURACY_VALUE',
'Maximum model space distance between geometric entities at asserted c
onnectivities');
#57841=UNCERTAINTY_MEASURE_WITH_UNIT(LENGTH_MEASURE(0.001),#57901,
'DISTANCE_ACCURACY_VALUE',
'Maximum model space distance between geometric entities at asserted c
onnectivities');
#57851=(
GEOMETRIC_REPRESENTATION_CONTEXT(3)
GLOBAL_UNCERTAINTY_ASSIGNED_CONTEXT((#57792))
GLOBAL_UNIT_ASSIGNED_CONTEXT((#57901,#57903,#57904))
REPRESENTATION_CONTEXT('','3D')
);
#57900=(
GEOMETRIC_REPRESENTATION_CONTEXT(3)
GLOBAL_UNCERTAINTY_ASSIGNED_CONTEXT((#57841))
GLOBAL_UNIT_ASSIGNED_CONTEXT((#57901,#57903,#57904))
REPRESENTATION_CONTEXT('','3D')
);
#57901=(
LENGTH_UNIT()
NAMED_UNIT(*)
SI_UNIT(.CENTI.,.METRE.)
);
#57903=(
NAMED_UNIT(*)
PLANE_ANGLE_UNIT()
SI_UNIT($,.RADIAN.)
);
#57904=(
NAMED_UNIT(*)
SI_UNIT($,.STERADIAN.)
SOLID_ANGLE_UNIT()
);
#57914=SHAPE_DEFINITION_REPRESENTATION(#57972,#58118);
#57972=PRODUCT_DEFINITION_SHAPE('',$,#58177);
#58118=SHAPE_REPRESENTATION('',(#14389),#57851);
#58167=PRODUCT_DEFINITION_CONTEXT('part definition',#58343,'design');
#58177=PRODUCT_DEFINITION('Indicator arm','Indicator arm',#58235,#58167);
#58235=PRODUCT_DEFINITION_FORMATION('',$,#58354);
#58343=APPLICATION_CONTEXT(
'Core Data for Automotive Mechanical Design Process');
#58344=PRODUCT_CONTEXT('part definition',#58343,'mechanical');
#58354=PRODUCT('Indicator arm','Indicator arm','Indicator arm',(#58344));
#58445=COLOUR_RGB('Light Blue',0.38,0.62,0.78);
#58446=FILL_AREA_STYLE_COLOUR('',#58445);
#58447=FILL_AREA_STYLE('',(#58446));
#58448=SURFACE_STYLE_FILL_AREA(#58447);
#58449=SURFACE_SIDE_STYLE('',(#58448));
#58450=SURFACE_STYLE_USAGE(.BOTH.,#58449);
#58451=PRESENTATION_STYLE_ASSIGNMENT((#58450));
ENDSEC;
END-ISO-10303-21;
